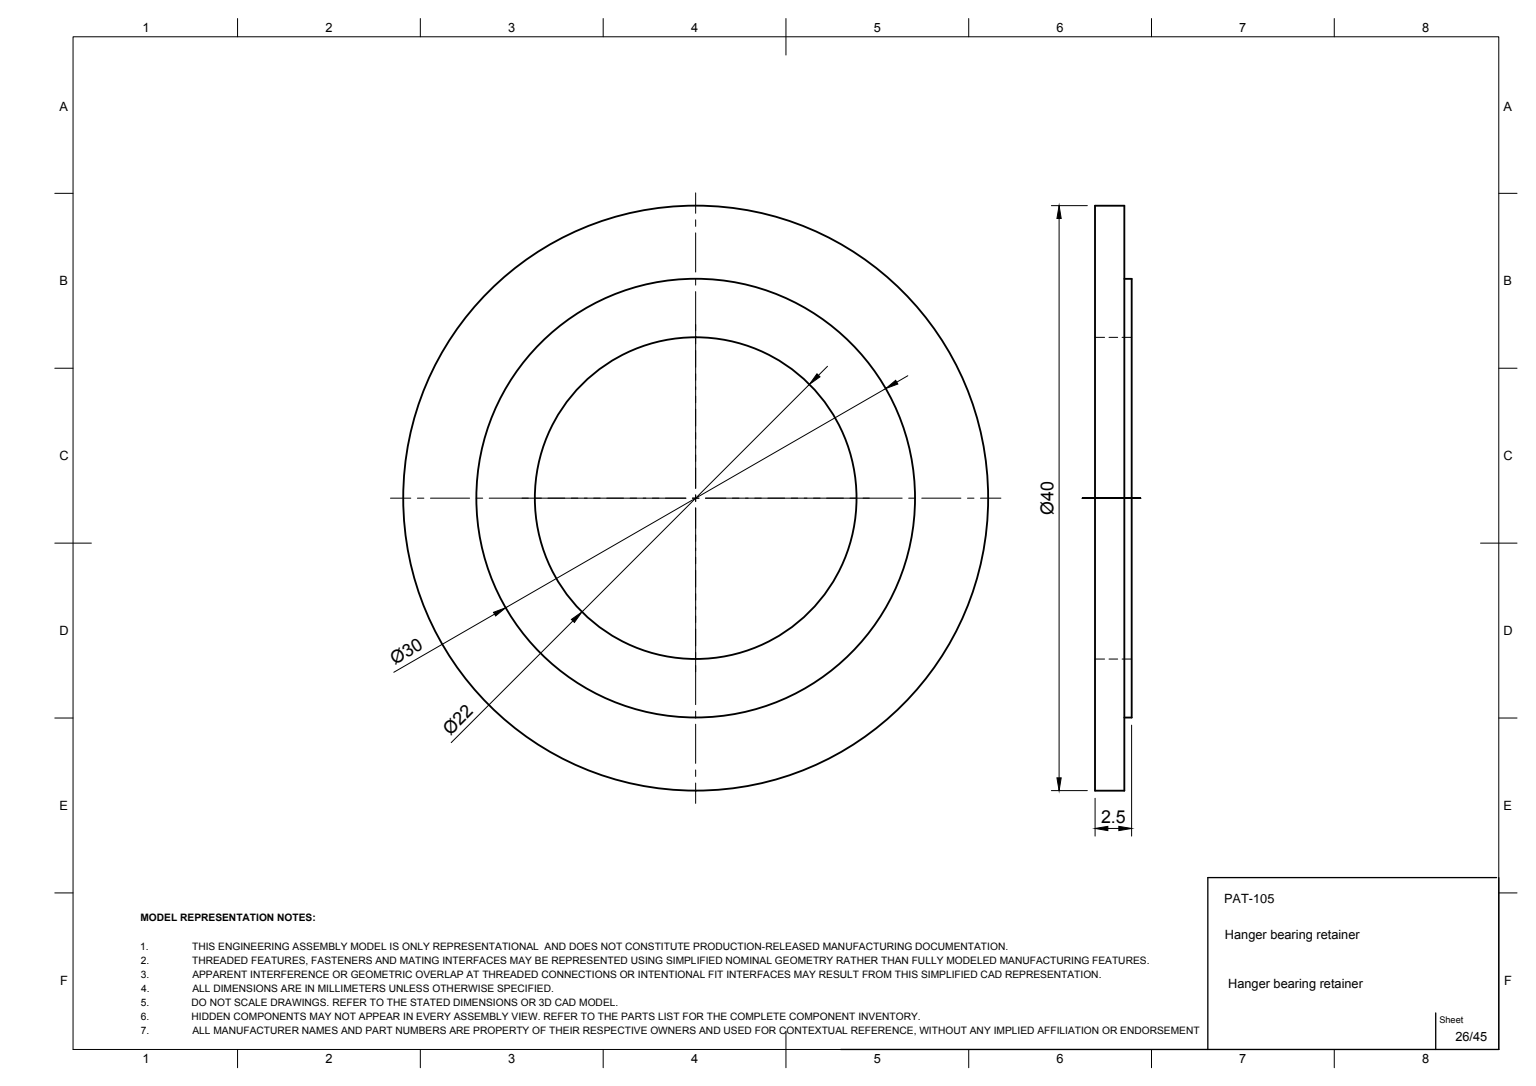
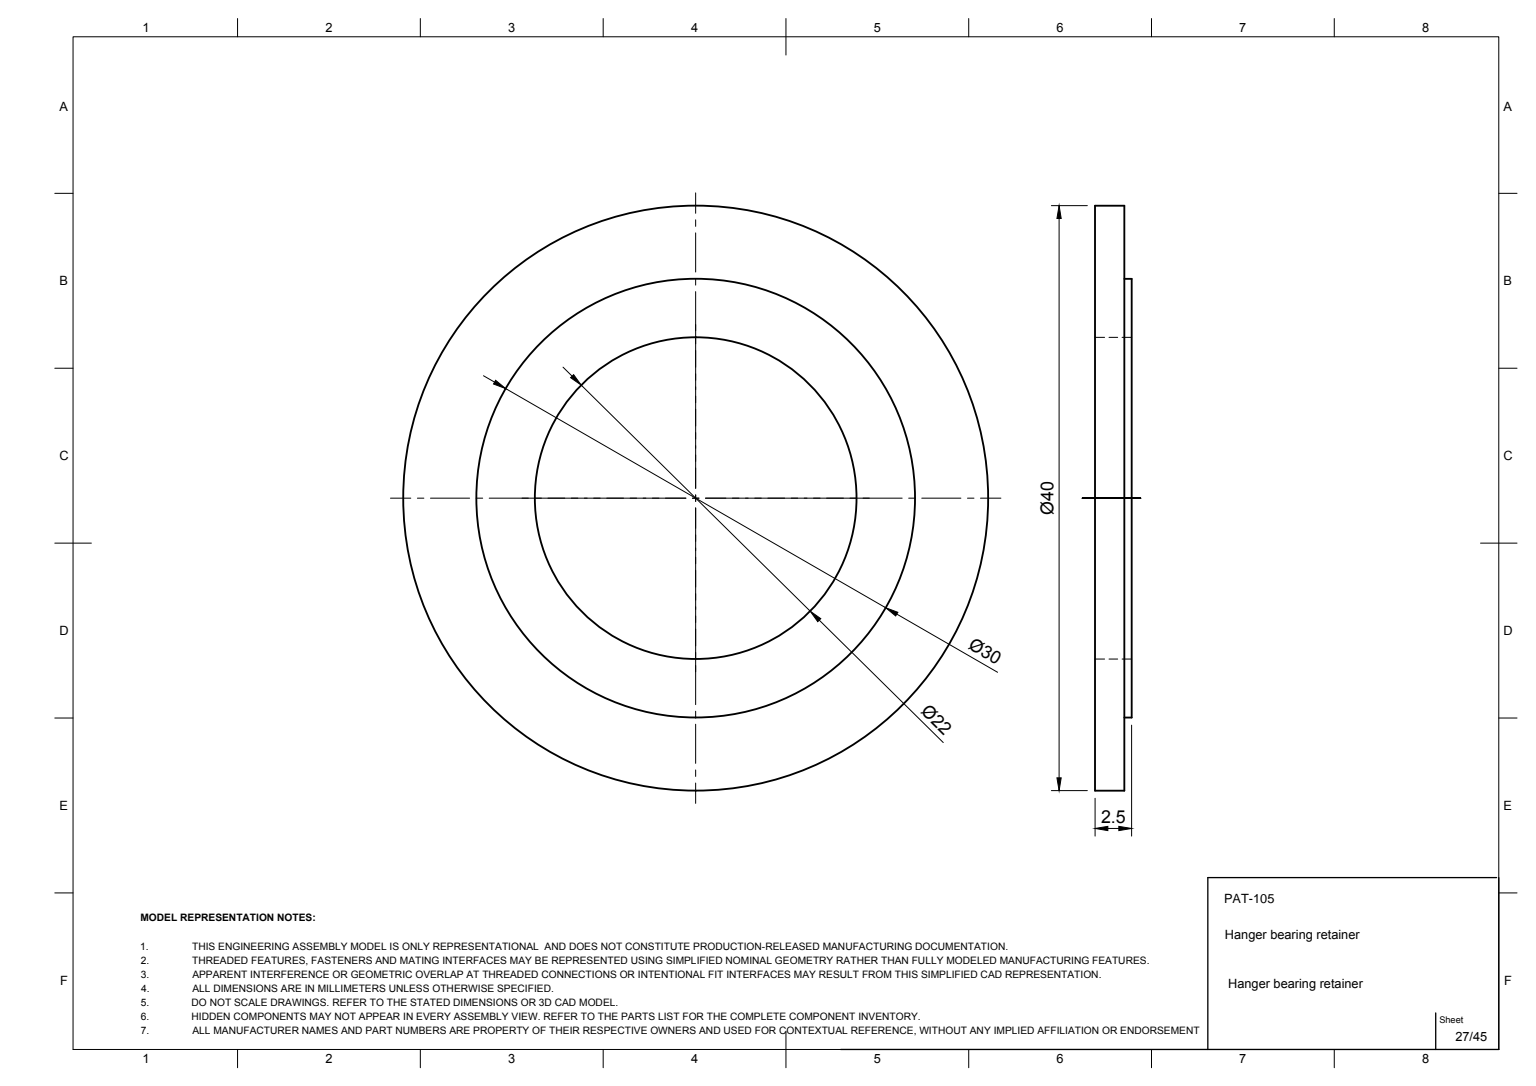
ISO-10303-21;
HEADER;
/* Generated by software containing ST-Developer
 * from STEP Tools, Inc. (www.steptools.com) 
 */

FILE_DESCRIPTION(
/* description */ ('Torque wrench calibration arm'),
/* implementation_level */ '2;1');

FILE_NAME(
/* name */ 'Hanger bearing retainer.step',
/* time_stamp */ '2026-10-28T03:24:52-07:00',
/* author */ (''),
/* organization */ (''),
/* preprocessor_version */ 'ST-DEVELOPER v20.2',
/* originating_system */ 'Autodesk Translation Framework v15.17.0.0',
/* authorisation */ '');

FILE_SCHEMA (('AUTOMOTIVE_DESIGN { 1 0 10303 214 3 1 1 }'));
ENDSEC;

DATA;
#10=MECHANICAL_DESIGN_GEOMETRIC_PRESENTATION_REPRESENTATION('',(#454),#12783);
#371=SHAPE_REPRESENTATION_RELATIONSHIP('SRR','None',#12954,#408);
#408=ADVANCED_BREP_SHAPE_REPRESENTATION('',(#506),#12763);
#454=STYLED_ITEM('',(#13212),#506);
#506=MANIFOLD_SOLID_BREP('Body1',#6525);
#615=FACE_BOUND('',#1606,.T.);
#616=FACE_BOUND('',#1610,.T.);
#617=FACE_BOUND('',#1612,.T.);
#796=PLANE('',#7487);
#797=PLANE('',#7494);
#798=PLANE('',#7495);
#1125=FACE_OUTER_BOUND('',#1604,.T.);
#1126=FACE_OUTER_BOUND('',#1605,.T.);
#1127=FACE_OUTER_BOUND('',#1607,.T.);
#1128=FACE_OUTER_BOUND('',#1608,.T.);
#1129=FACE_OUTER_BOUND('',#1609,.T.);
#1130=FACE_OUTER_BOUND('',#1611,.T.);
#1604=EDGE_LOOP('',(#5425,#5426,#5427,#5428));
#1605=EDGE_LOOP('',(#5429));
#1606=EDGE_LOOP('',(#5430));
#1607=EDGE_LOOP('',(#5431,#5432,#5433,#5434));
#1608=EDGE_LOOP('',(#5435,#5436,#5437,#5438));
#1609=EDGE_LOOP('',(#5439));
#1610=EDGE_LOOP('',(#5440));
#1611=EDGE_LOOP('',(#5441));
#1612=EDGE_LOOP('',(#5442));
#2069=LINE('',#11691,#2484);
#2070=LINE('',#11698,#2485);
#2071=LINE('',#11704,#2486);
#2484=VECTOR('',#9145,1.5);
#2485=VECTOR('',#9154,1.1);
#2486=VECTOR('',#9161,2.);
#2840=CIRCLE('',#7485,1.5);
#2841=CIRCLE('',#7486,1.5);
#2842=CIRCLE('',#7488,1.1);
#2843=CIRCLE('',#7490,1.1);
#2844=CIRCLE('',#7492,2.);
#2845=CIRCLE('',#7493,2.);
#3338=VERTEX_POINT('',#11688);
#3339=VERTEX_POINT('',#11690);
#3340=VERTEX_POINT('',#11694);
#3341=VERTEX_POINT('',#11697);
#3342=VERTEX_POINT('',#11701);
#3343=VERTEX_POINT('',#11703);
#4070=EDGE_CURVE('',#3338,#3338,#2840,.T.);
#4071=EDGE_CURVE('',#3338,#3339,#2069,.T.);
#4072=EDGE_CURVE('',#3339,#3339,#2841,.T.);
#4073=EDGE_CURVE('',#3340,#3340,#2842,.T.);
#4074=EDGE_CURVE('',#3340,#3341,#2070,.T.);
#4075=EDGE_CURVE('',#3341,#3341,#2843,.T.);
#4076=EDGE_CURVE('',#3342,#3342,#2844,.T.);
#4077=EDGE_CURVE('',#3342,#3343,#2071,.T.);
#4078=EDGE_CURVE('',#3343,#3343,#2845,.T.);
#5425=ORIENTED_EDGE('',*,*,#4070,.F.);
#5426=ORIENTED_EDGE('',*,*,#4071,.T.);
#5427=ORIENTED_EDGE('',*,*,#4072,.F.);
#5428=ORIENTED_EDGE('',*,*,#4071,.F.);
#5429=ORIENTED_EDGE('',*,*,#4070,.T.);
#5430=ORIENTED_EDGE('',*,*,#4073,.T.);
#5431=ORIENTED_EDGE('',*,*,#4073,.F.);
#5432=ORIENTED_EDGE('',*,*,#4074,.T.);
#5433=ORIENTED_EDGE('',*,*,#4075,.T.);
#5434=ORIENTED_EDGE('',*,*,#4074,.F.);
#5435=ORIENTED_EDGE('',*,*,#4076,.F.);
#5436=ORIENTED_EDGE('',*,*,#4077,.T.);
#5437=ORIENTED_EDGE('',*,*,#4078,.T.);
#5438=ORIENTED_EDGE('',*,*,#4077,.F.);
#5439=ORIENTED_EDGE('',*,*,#4076,.T.);
#5440=ORIENTED_EDGE('',*,*,#4072,.T.);
#5441=ORIENTED_EDGE('',*,*,#4078,.F.);
#5442=ORIENTED_EDGE('',*,*,#4075,.F.);
#6061=CYLINDRICAL_SURFACE('',#7484,1.5);
#6062=CYLINDRICAL_SURFACE('',#7489,1.1);
#6063=CYLINDRICAL_SURFACE('',#7491,2.);
#6350=ADVANCED_FACE('',(#1125),#6061,.T.);
#6351=ADVANCED_FACE('',(#1126,#615),#796,.T.);
#6352=ADVANCED_FACE('',(#1127),#6062,.F.);
#6353=ADVANCED_FACE('',(#1128),#6063,.T.);
#6354=ADVANCED_FACE('',(#1129,#616),#797,.T.);
#6355=ADVANCED_FACE('',(#1130,#617),#798,.F.);
#6525=CLOSED_SHELL('',(#6350,#6351,#6352,#6353,#6354,#6355));
#7483=AXIS2_PLACEMENT_3D('',#11686,#9139,#9140);
#7484=AXIS2_PLACEMENT_3D('',#11687,#9141,#9142);
#7485=AXIS2_PLACEMENT_3D('',#11689,#9143,#9144);
#7486=AXIS2_PLACEMENT_3D('',#11692,#9146,#9147);
#7487=AXIS2_PLACEMENT_3D('',#11693,#9148,#9149);
#7488=AXIS2_PLACEMENT_3D('',#11695,#9150,#9151);
#7489=AXIS2_PLACEMENT_3D('',#11696,#9152,#9153);
#7490=AXIS2_PLACEMENT_3D('',#11699,#9155,#9156);
#7491=AXIS2_PLACEMENT_3D('',#11700,#9157,#9158);
#7492=AXIS2_PLACEMENT_3D('',#11702,#9159,#9160);
#7493=AXIS2_PLACEMENT_3D('',#11705,#9162,#9163);
#7494=AXIS2_PLACEMENT_3D('',#11706,#9164,#9165);
#7495=AXIS2_PLACEMENT_3D('',#11707,#9166,#9167);
#9139=DIRECTION('axis',(0.,0.,1.));
#9140=DIRECTION('refdir',(1.,0.,0.));
#9141=DIRECTION('center_axis',(0.,1.,0.));
#9142=DIRECTION('ref_axis',(1.,0.,0.));
#9143=DIRECTION('center_axis',(0.,1.,0.));
#9144=DIRECTION('ref_axis',(1.,0.,0.));
#9145=DIRECTION('',(0.,-1.,0.));
#9146=DIRECTION('center_axis',(0.,-1.,0.));
#9147=DIRECTION('ref_axis',(1.,0.,0.));
#9148=DIRECTION('center_axis',(0.,1.,0.));
#9149=DIRECTION('ref_axis',(1.,0.,0.));
#9150=DIRECTION('center_axis',(0.,-1.,0.));
#9151=DIRECTION('ref_axis',(1.,0.,0.));
#9152=DIRECTION('center_axis',(0.,1.,0.));
#9153=DIRECTION('ref_axis',(1.,0.,0.));
#9154=DIRECTION('',(0.,-1.,0.));
#9155=DIRECTION('center_axis',(0.,-1.,0.));
#9156=DIRECTION('ref_axis',(1.,0.,0.));
#9157=DIRECTION('center_axis',(0.,1.,0.));
#9158=DIRECTION('ref_axis',(1.,0.,0.));
#9159=DIRECTION('center_axis',(0.,1.,0.));
#9160=DIRECTION('ref_axis',(1.,0.,0.));
#9161=DIRECTION('',(0.,-1.,0.));
#9162=DIRECTION('center_axis',(0.,1.,0.));
#9163=DIRECTION('ref_axis',(1.,0.,0.));
#9164=DIRECTION('center_axis',(0.,1.,0.));
#9165=DIRECTION('ref_axis',(1.,0.,0.));
#9166=DIRECTION('center_axis',(0.,1.,0.));
#9167=DIRECTION('ref_axis',(1.,0.,0.));
#11686=CARTESIAN_POINT('',(0.,0.,0.));
#11687=CARTESIAN_POINT('Origin',(50.,8.,8.));
#11688=CARTESIAN_POINT('',(48.5,8.05,8.));
#11689=CARTESIAN_POINT('Origin',(50.,8.05,8.));
#11690=CARTESIAN_POINT('',(48.5,8.,8.));
#11691=CARTESIAN_POINT('',(48.5,8.,8.));
#11692=CARTESIAN_POINT('Origin',(50.,8.,8.));
#11693=CARTESIAN_POINT('Origin',(50.,8.05,8.));
#11694=CARTESIAN_POINT('',(48.9,8.05,8.));
#11695=CARTESIAN_POINT('Origin',(50.,8.05,8.));
#11696=CARTESIAN_POINT('Origin',(50.,7.8,8.));
#11697=CARTESIAN_POINT('',(48.9,7.8,8.));
#11698=CARTESIAN_POINT('',(48.9,7.8,8.));
#11699=CARTESIAN_POINT('Origin',(50.,7.8,8.));
#11700=CARTESIAN_POINT('Origin',(50.,7.8,8.));
#11701=CARTESIAN_POINT('',(48.,8.,8.));
#11702=CARTESIAN_POINT('Origin',(50.,8.,8.));
#11703=CARTESIAN_POINT('',(48.,7.8,8.));
#11704=CARTESIAN_POINT('',(48.,7.8,8.));
#11705=CARTESIAN_POINT('Origin',(50.,7.8,8.));
#11706=CARTESIAN_POINT('Origin',(50.,8.,8.));
#11707=CARTESIAN_POINT('Origin',(50.,7.8,8.));
#12719=UNCERTAINTY_MEASURE_WITH_UNIT(LENGTH_MEASURE(0.001),#12784,
'DISTANCE_ACCURACY_VALUE',
'Maximum model space distance between geometric entities at asserted c
onnectivities');
#12739=UNCERTAINTY_MEASURE_WITH_UNIT(LENGTH_MEASURE(0.001),#12784,
'DISTANCE_ACCURACY_VALUE',
'Maximum model space distance between geometric entities at asserted c
onnectivities');
#12763=(
GEOMETRIC_REPRESENTATION_CONTEXT(3)
GLOBAL_UNCERTAINTY_ASSIGNED_CONTEXT((#12719))
GLOBAL_UNIT_ASSIGNED_CONTEXT((#12784,#12786,#12787))
REPRESENTATION_CONTEXT('','3D')
);
#12783=(
GEOMETRIC_REPRESENTATION_CONTEXT(3)
GLOBAL_UNCERTAINTY_ASSIGNED_CONTEXT((#12739))
GLOBAL_UNIT_ASSIGNED_CONTEXT((#12784,#12786,#12787))
REPRESENTATION_CONTEXT('','3D')
);
#12784=(
LENGTH_UNIT()
NAMED_UNIT(*)
SI_UNIT(.CENTI.,.METRE.)
);
#12786=(
NAMED_UNIT(*)
PLANE_ANGLE_UNIT()
SI_UNIT($,.RADIAN.)
);
#12787=(
NAMED_UNIT(*)
SI_UNIT($,.STERADIAN.)
SOLID_ANGLE_UNIT()
);
#12811=SHAPE_DEFINITION_REPRESENTATION(#12880,#12954);
#12880=PRODUCT_DEFINITION_SHAPE('',$,#12998);
#12954=SHAPE_REPRESENTATION('',(#7483),#12763);
#12974=PRODUCT_DEFINITION_CONTEXT('part definition',#13105,'design');
#12998=PRODUCT_DEFINITION('Hanger bearing retainer',
'Hanger bearing retainer',#13041,#12974);
#13041=PRODUCT_DEFINITION_FORMATION('',$,#13130);
#13105=APPLICATION_CONTEXT(
'Core Data for Automotive Mechanical Design Process');
#13106=PRODUCT_CONTEXT('part definition',#13105,'mechanical');
#13130=PRODUCT('Hanger bearing retainer','Hanger bearing retainer',
'Hanger bearing retainer',(#13106));
#13206=COLOUR_RGB('Grey',0.48,0.52,0.57);
#13207=FILL_AREA_STYLE_COLOUR('',#13206);
#13208=FILL_AREA_STYLE('',(#13207));
#13209=SURFACE_STYLE_FILL_AREA(#13208);
#13210=SURFACE_SIDE_STYLE('',(#13209));
#13211=SURFACE_STYLE_USAGE(.BOTH.,#13210);
#13212=PRESENTATION_STYLE_ASSIGNMENT((#13211));
ENDSEC;
END-ISO-10303-21;
